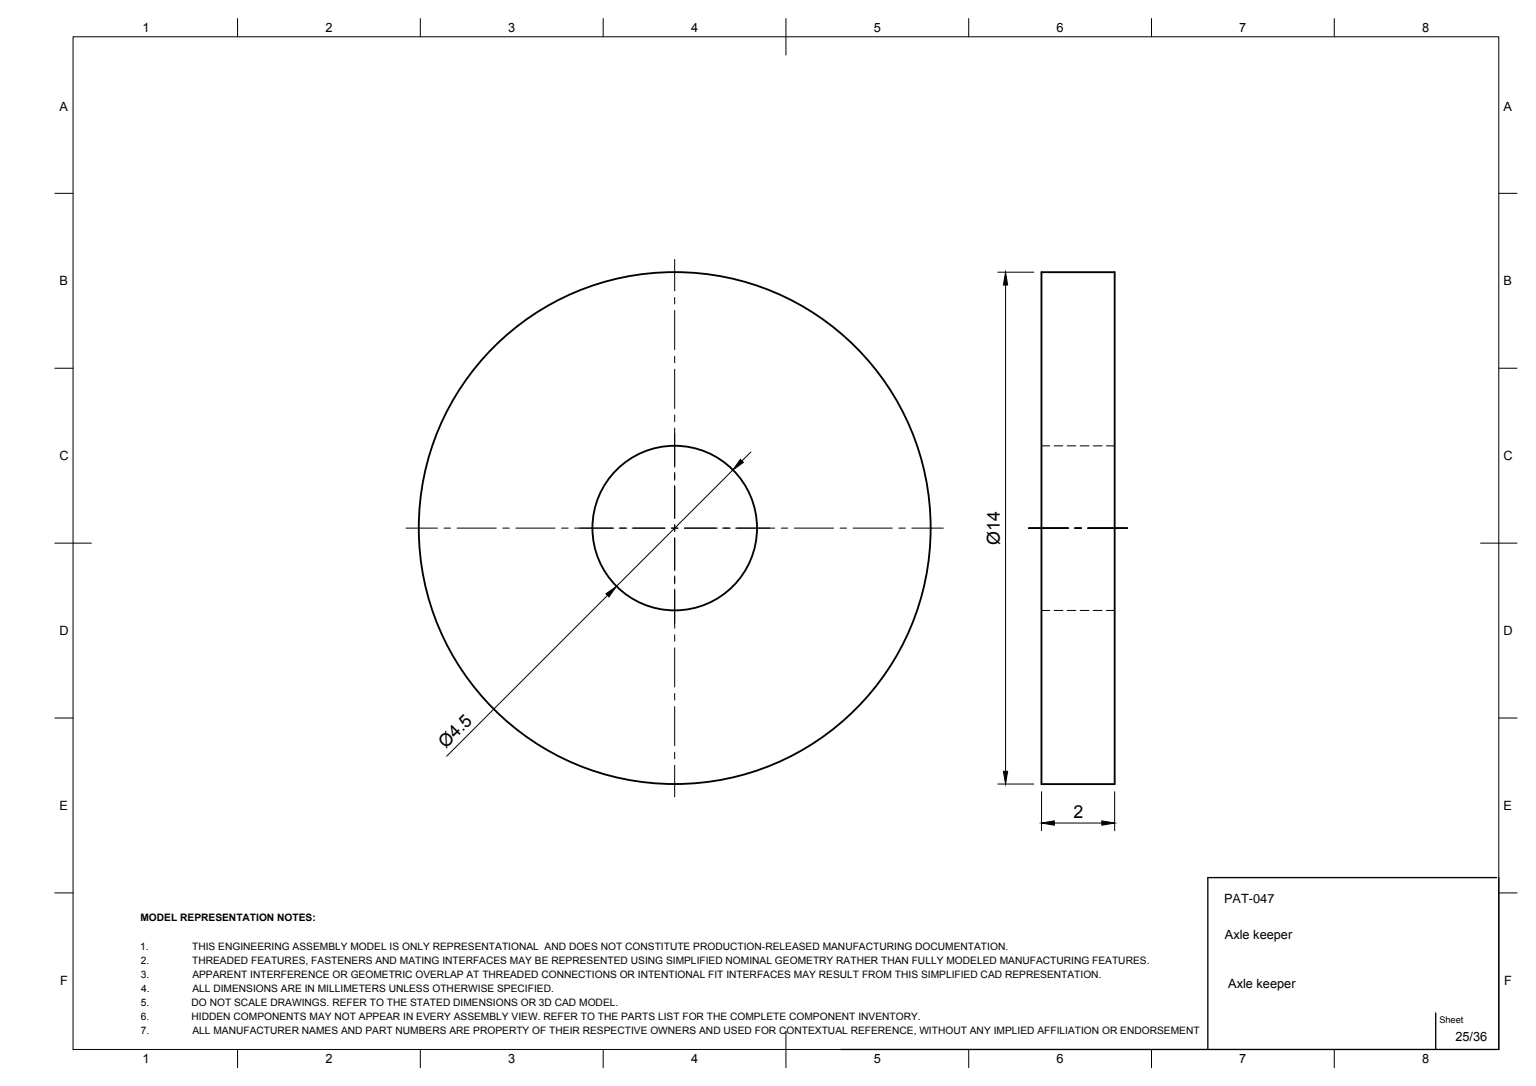
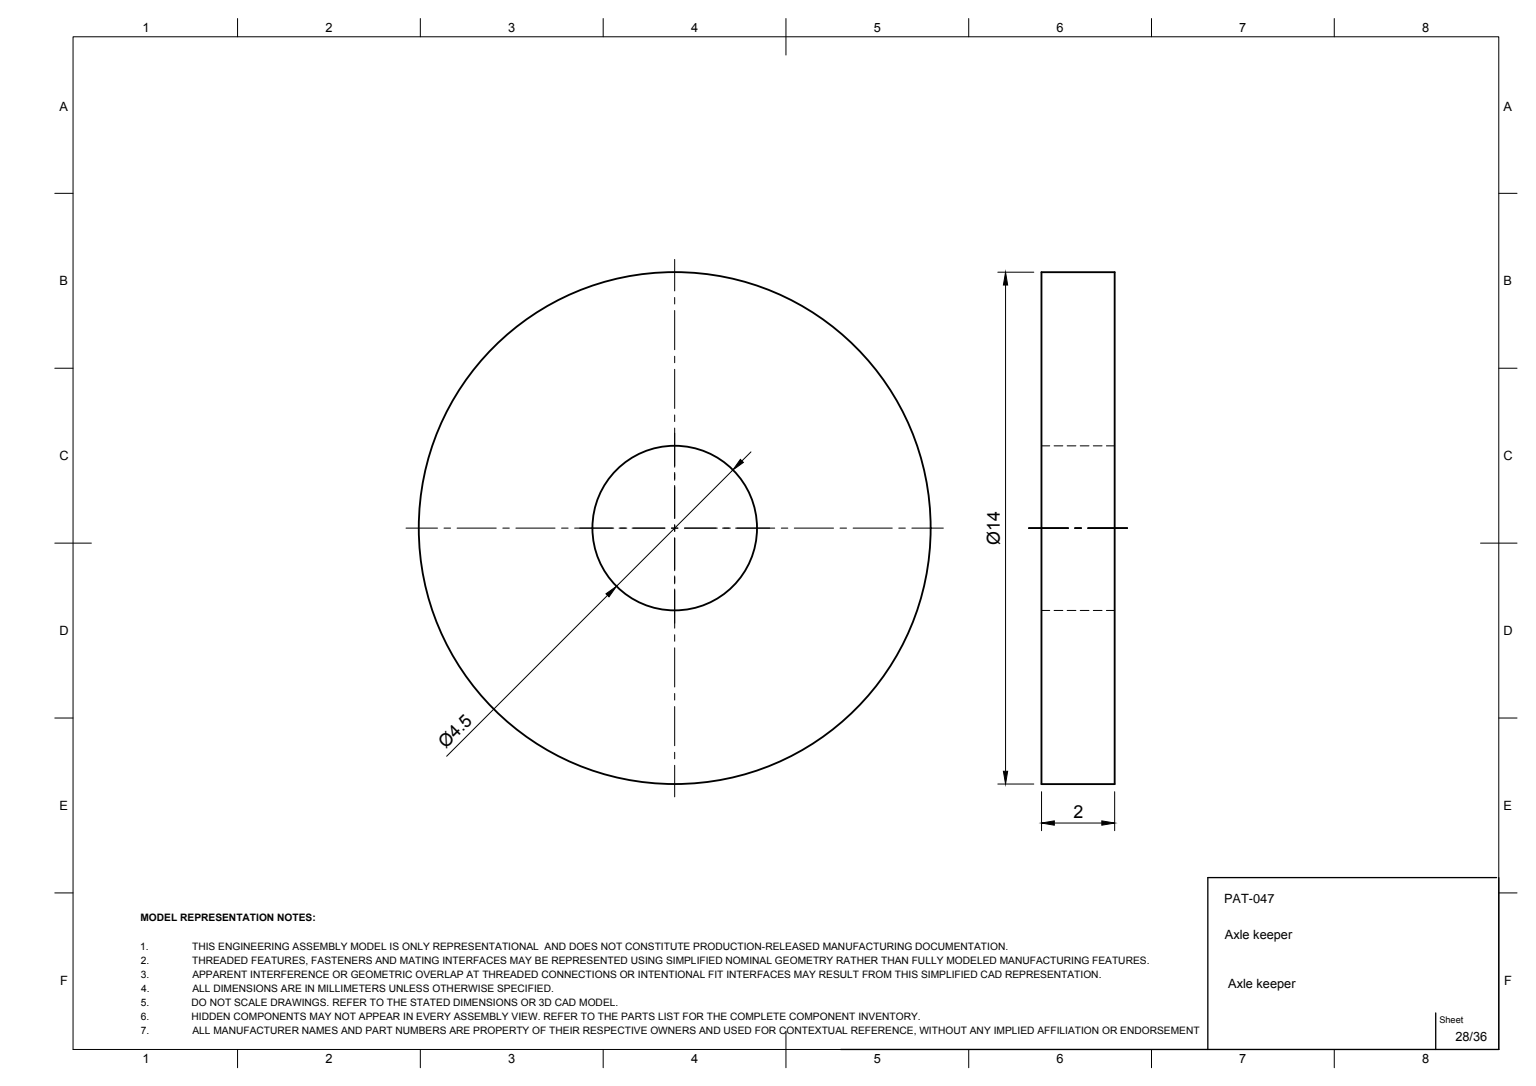
ISO-10303-21;
HEADER;
/* Generated by software containing ST-Developer
 * from STEP Tools, Inc. (www.steptools.com) 
 */

FILE_DESCRIPTION(
/* description */ ('Gravity roller conveyor section'),
/* implementation_level */ '2;1');

FILE_NAME(
/* name */ 'Axle keeper.step',
/* time_stamp */ '2026-11-02T07:43:02-08:00',
/* author */ (''),
/* organization */ (''),
/* preprocessor_version */ 'ST-DEVELOPER v20.2',
/* originating_system */ 'Autodesk Translation Framework v15.17.0.0',
/* authorisation */ '');

FILE_SCHEMA (('AUTOMOTIVE_DESIGN { 1 0 10303 214 3 1 1 }'));
ENDSEC;

DATA;
#10=MECHANICAL_DESIGN_GEOMETRIC_PRESENTATION_REPRESENTATION('',(#550),#13821);
#482=SHAPE_REPRESENTATION_RELATIONSHIP('SRR','None',#14020,#516);
#516=ADVANCED_BREP_SHAPE_REPRESENTATION('',(#590),#13807);
#550=STYLED_ITEM('',(#14192),#590);
#590=MANIFOLD_SOLID_BREP('Body1',#7650);
#674=FACE_BOUND('',#1787,.T.);
#675=FACE_BOUND('',#1789,.T.);
#939=PLANE('',#8472);
#940=PLANE('',#8473);
#1300=FACE_OUTER_BOUND('',#1784,.T.);
#1301=FACE_OUTER_BOUND('',#1785,.T.);
#1302=FACE_OUTER_BOUND('',#1786,.T.);
#1303=FACE_OUTER_BOUND('',#1788,.T.);
#1784=EDGE_LOOP('',(#6618,#6619,#6620,#6621));
#1785=EDGE_LOOP('',(#6622,#6623,#6624,#6625));
#1786=EDGE_LOOP('',(#6626));
#1787=EDGE_LOOP('',(#6627));
#1788=EDGE_LOOP('',(#6628));
#1789=EDGE_LOOP('',(#6629));
#2536=LINE('',#12743,#3254);
#2537=LINE('',#12749,#3255);
#3254=VECTOR('',#10255,0.225);
#3255=VECTOR('',#10262,0.7);
#3474=CIRCLE('',#8467,0.225);
#3475=CIRCLE('',#8468,0.225);
#3476=CIRCLE('',#8470,0.7);
#3477=CIRCLE('',#8471,0.7);
#4060=VERTEX_POINT('',#12740);
#4061=VERTEX_POINT('',#12742);
#4062=VERTEX_POINT('',#12746);
#4063=VERTEX_POINT('',#12748);
#4946=EDGE_CURVE('',#4060,#4060,#3474,.T.);
#4947=EDGE_CURVE('',#4060,#4061,#2536,.T.);
#4948=EDGE_CURVE('',#4061,#4061,#3475,.T.);
#4949=EDGE_CURVE('',#4062,#4062,#3476,.T.);
#4950=EDGE_CURVE('',#4062,#4063,#2537,.T.);
#4951=EDGE_CURVE('',#4063,#4063,#3477,.T.);
#6618=ORIENTED_EDGE('',*,*,#4946,.F.);
#6619=ORIENTED_EDGE('',*,*,#4947,.T.);
#6620=ORIENTED_EDGE('',*,*,#4948,.T.);
#6621=ORIENTED_EDGE('',*,*,#4947,.F.);
#6622=ORIENTED_EDGE('',*,*,#4949,.F.);
#6623=ORIENTED_EDGE('',*,*,#4950,.T.);
#6624=ORIENTED_EDGE('',*,*,#4951,.T.);
#6625=ORIENTED_EDGE('',*,*,#4950,.F.);
#6626=ORIENTED_EDGE('',*,*,#4949,.T.);
#6627=ORIENTED_EDGE('',*,*,#4946,.T.);
#6628=ORIENTED_EDGE('',*,*,#4951,.F.);
#6629=ORIENTED_EDGE('',*,*,#4948,.F.);
#7178=CYLINDRICAL_SURFACE('',#8466,0.225);
#7179=CYLINDRICAL_SURFACE('',#8469,0.7);
#7501=ADVANCED_FACE('',(#1300),#7178,.F.);
#7502=ADVANCED_FACE('',(#1301),#7179,.T.);
#7503=ADVANCED_FACE('',(#1302,#674),#939,.T.);
#7504=ADVANCED_FACE('',(#1303,#675),#940,.F.);
#7650=CLOSED_SHELL('',(#7501,#7502,#7503,#7504));
#8465=AXIS2_PLACEMENT_3D('',#12738,#10249,#10250);
#8466=AXIS2_PLACEMENT_3D('',#12739,#10251,#10252);
#8467=AXIS2_PLACEMENT_3D('',#12741,#10253,#10254);
#8468=AXIS2_PLACEMENT_3D('',#12744,#10256,#10257);
#8469=AXIS2_PLACEMENT_3D('',#12745,#10258,#10259);
#8470=AXIS2_PLACEMENT_3D('',#12747,#10260,#10261);
#8471=AXIS2_PLACEMENT_3D('',#12750,#10263,#10264);
#8472=AXIS2_PLACEMENT_3D('',#12751,#10265,#10266);
#8473=AXIS2_PLACEMENT_3D('',#12752,#10267,#10268);
#10249=DIRECTION('axis',(0.,0.,1.));
#10250=DIRECTION('refdir',(1.,0.,0.));
#10251=DIRECTION('center_axis',(0.,1.,0.));
#10252=DIRECTION('ref_axis',(1.,0.,0.));
#10253=DIRECTION('center_axis',(0.,-1.,0.));
#10254=DIRECTION('ref_axis',(1.,0.,0.));
#10255=DIRECTION('',(0.,-1.,0.));
#10256=DIRECTION('center_axis',(0.,-1.,0.));
#10257=DIRECTION('ref_axis',(1.,0.,0.));
#10258=DIRECTION('center_axis',(0.,1.,0.));
#10259=DIRECTION('ref_axis',(1.,0.,0.));
#10260=DIRECTION('center_axis',(0.,1.,0.));
#10261=DIRECTION('ref_axis',(1.,0.,0.));
#10262=DIRECTION('',(0.,-1.,0.));
#10263=DIRECTION('center_axis',(0.,1.,0.));
#10264=DIRECTION('ref_axis',(1.,0.,0.));
#10265=DIRECTION('center_axis',(0.,1.,0.));
#10266=DIRECTION('ref_axis',(1.,0.,0.));
#10267=DIRECTION('center_axis',(0.,1.,0.));
#10268=DIRECTION('ref_axis',(1.,0.,0.));
#12738=CARTESIAN_POINT('',(0.,0.,0.));
#12739=CARTESIAN_POINT('Origin',(3.,-3.2,8.));
#12740=CARTESIAN_POINT('',(2.775,-3.,8.));
#12741=CARTESIAN_POINT('Origin',(3.,-3.,8.));
#12742=CARTESIAN_POINT('',(2.775,-3.2,8.));
#12743=CARTESIAN_POINT('',(2.775,-3.2,8.));
#12744=CARTESIAN_POINT('Origin',(3.,-3.2,8.));
#12745=CARTESIAN_POINT('Origin',(3.,-3.2,8.));
#12746=CARTESIAN_POINT('',(2.3,-3.,8.));
#12747=CARTESIAN_POINT('Origin',(3.,-3.,8.));
#12748=CARTESIAN_POINT('',(2.3,-3.2,8.));
#12749=CARTESIAN_POINT('',(2.3,-3.2,8.));
#12750=CARTESIAN_POINT('Origin',(3.,-3.2,8.));
#12751=CARTESIAN_POINT('Origin',(3.,-3.,8.));
#12752=CARTESIAN_POINT('Origin',(3.,-3.2,8.));
#13768=UNCERTAINTY_MEASURE_WITH_UNIT(LENGTH_MEASURE(0.001),#13822,
'DISTANCE_ACCURACY_VALUE',
'Maximum model space distance between geometric entities at asserted c
onnectivities');
#13782=UNCERTAINTY_MEASURE_WITH_UNIT(LENGTH_MEASURE(0.001),#13822,
'DISTANCE_ACCURACY_VALUE',
'Maximum model space distance between geometric entities at asserted c
onnectivities');
#13807=(
GEOMETRIC_REPRESENTATION_CONTEXT(3)
GLOBAL_UNCERTAINTY_ASSIGNED_CONTEXT((#13768))
GLOBAL_UNIT_ASSIGNED_CONTEXT((#13822,#13824,#13825))
REPRESENTATION_CONTEXT('','3D')
);
#13821=(
GEOMETRIC_REPRESENTATION_CONTEXT(3)
GLOBAL_UNCERTAINTY_ASSIGNED_CONTEXT((#13782))
GLOBAL_UNIT_ASSIGNED_CONTEXT((#13822,#13824,#13825))
REPRESENTATION_CONTEXT('','3D')
);
#13822=(
LENGTH_UNIT()
NAMED_UNIT(*)
SI_UNIT(.CENTI.,.METRE.)
);
#13824=(
NAMED_UNIT(*)
PLANE_ANGLE_UNIT()
SI_UNIT($,.RADIAN.)
);
#13825=(
NAMED_UNIT(*)
SI_UNIT($,.STERADIAN.)
SOLID_ANGLE_UNIT()
);
#13850=SHAPE_DEFINITION_REPRESENTATION(#13888,#14020);
#13888=PRODUCT_DEFINITION_SHAPE('',$,#14059);
#14020=SHAPE_REPRESENTATION('',(#8465),#13807);
#14034=PRODUCT_DEFINITION_CONTEXT('part definition',#14150,'design');
#14059=PRODUCT_DEFINITION('Axle keeper','Axle keeper',#14097,#14034);
#14097=PRODUCT_DEFINITION_FORMATION('',$,#14176);
#14150=APPLICATION_CONTEXT(
'Core Data for Automotive Mechanical Design Process');
#14151=PRODUCT_CONTEXT('part definition',#14150,'mechanical');
#14176=PRODUCT('Axle keeper','Axle keeper','Axle keeper',(#14151));
#14192=PRESENTATION_STYLE_ASSIGNMENT((#14197));
#14197=SURFACE_STYLE_USAGE(.BOTH.,#14202);
#14202=SURFACE_SIDE_STYLE('',(#14207));
#14207=SURFACE_STYLE_FILL_AREA(#14212);
#14212=FILL_AREA_STYLE('CAD Library Painted - Engineering blue',(#14217));
#14217=FILL_AREA_STYLE_COLOUR('CAD Library Painted - Engineering blue',
#14222);
#14222=COLOUR_RGB('CAD Library Painted - Engineering blue',0.12156862745098,
0.356862745098039,0.6);
ENDSEC;
END-ISO-10303-21;
